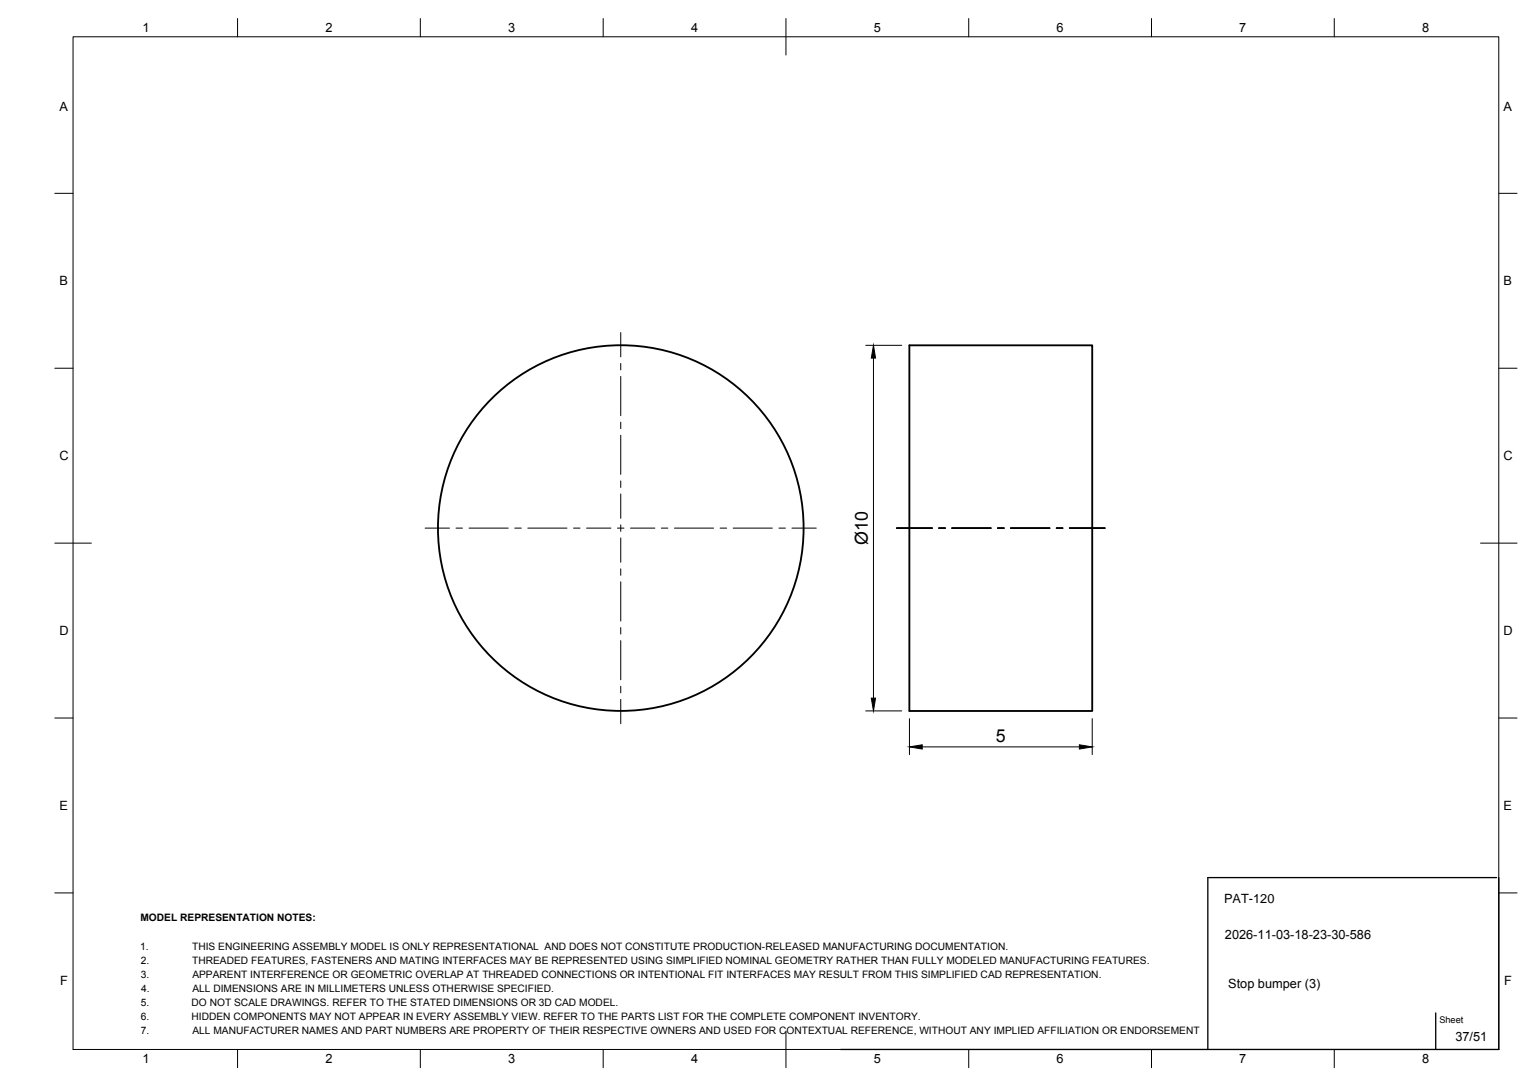
ISO-10303-21;
HEADER;
/* Generated by software containing ST-Developer
 * from STEP Tools, Inc. (www.steptools.com) 
 */

FILE_DESCRIPTION(
/* description */ ('Vibration shaker table dummy'),
/* implementation_level */ '2;1');

FILE_NAME(
/* name */ 'Stop bumper (3).step',
/* time_stamp */ '2026-10-27T10:55:14-07:00',
/* author */ (''),
/* organization */ (''),
/* preprocessor_version */ 'ST-DEVELOPER v20.2',
/* originating_system */ 'Autodesk Translation Framework v15.17.0.0',
/* authorisation */ '');

FILE_SCHEMA (('AUTOMOTIVE_DESIGN { 1 0 10303 214 3 1 1 }'));
ENDSEC;

DATA;
#10=MECHANICAL_DESIGN_GEOMETRIC_PRESENTATION_REPRESENTATION('',(#718),#22394);
#626=SHAPE_REPRESENTATION_RELATIONSHIP('SRR','None',#22672,#672);
#672=ADVANCED_BREP_SHAPE_REPRESENTATION('',(#764),#22378);
#718=STYLED_ITEM('',(#22975),#764);
#764=MANIFOLD_SOLID_BREP('Body1',#9236);
#1230=PLANE('',#10337);
#1231=PLANE('',#10338);
#1630=FACE_OUTER_BOUND('',#2300,.T.);
#1631=FACE_OUTER_BOUND('',#2301,.T.);
#1632=FACE_OUTER_BOUND('',#2302,.T.);
#2300=EDGE_LOOP('',(#7488,#7489,#7490,#7491));
#2301=EDGE_LOOP('',(#7492));
#2302=EDGE_LOOP('',(#7493));
#2985=LINE('',#21090,#3604);
#3604=VECTOR('',#12465,0.5);
#4114=CIRCLE('',#10335,0.5);
#4115=CIRCLE('',#10336,0.5);
#4781=VERTEX_POINT('',#21087);
#4782=VERTEX_POINT('',#21089);
#5737=EDGE_CURVE('',#4781,#4781,#4114,.T.);
#5738=EDGE_CURVE('',#4781,#4782,#2985,.T.);
#5739=EDGE_CURVE('',#4782,#4782,#4115,.T.);
#7488=ORIENTED_EDGE('',*,*,#5737,.F.);
#7489=ORIENTED_EDGE('',*,*,#5738,.T.);
#7490=ORIENTED_EDGE('',*,*,#5739,.T.);
#7491=ORIENTED_EDGE('',*,*,#5738,.F.);
#7492=ORIENTED_EDGE('',*,*,#5737,.T.);
#7493=ORIENTED_EDGE('',*,*,#5739,.F.);
#8621=CYLINDRICAL_SURFACE('',#10334,0.5);
#8995=ADVANCED_FACE('',(#1630),#8621,.T.);
#8996=ADVANCED_FACE('',(#1631),#1230,.T.);
#8997=ADVANCED_FACE('',(#1632),#1231,.F.);
#9236=CLOSED_SHELL('',(#8995,#8996,#8997));
#10333=AXIS2_PLACEMENT_3D('',#21085,#12459,#12460);
#10334=AXIS2_PLACEMENT_3D('',#21086,#12461,#12462);
#10335=AXIS2_PLACEMENT_3D('',#21088,#12463,#12464);
#10336=AXIS2_PLACEMENT_3D('',#21091,#12466,#12467);
#10337=AXIS2_PLACEMENT_3D('',#21092,#12468,#12469);
#10338=AXIS2_PLACEMENT_3D('',#21093,#12470,#12471);
#12459=DIRECTION('axis',(0.,0.,1.));
#12460=DIRECTION('refdir',(1.,0.,0.));
#12461=DIRECTION('center_axis',(0.,0.,1.));
#12462=DIRECTION('ref_axis',(1.,0.,0.));
#12463=DIRECTION('center_axis',(0.,0.,1.));
#12464=DIRECTION('ref_axis',(1.,0.,0.));
#12465=DIRECTION('',(0.,0.,-1.));
#12466=DIRECTION('center_axis',(0.,0.,1.));
#12467=DIRECTION('ref_axis',(1.,0.,0.));
#12468=DIRECTION('center_axis',(0.,0.,1.));
#12469=DIRECTION('ref_axis',(1.,0.,0.));
#12470=DIRECTION('center_axis',(0.,0.,1.));
#12471=DIRECTION('ref_axis',(1.,0.,0.));
#21085=CARTESIAN_POINT('',(0.,0.,0.));
#21086=CARTESIAN_POINT('Origin',(0.,6.,17.3));
#21087=CARTESIAN_POINT('',(-0.5,6.,17.8));
#21088=CARTESIAN_POINT('Origin',(0.,6.,17.8));
#21089=CARTESIAN_POINT('',(-0.5,6.,17.3));
#21090=CARTESIAN_POINT('',(-0.5,6.,17.3));
#21091=CARTESIAN_POINT('Origin',(0.,6.,17.3));
#21092=CARTESIAN_POINT('Origin',(0.,6.,17.8));
#21093=CARTESIAN_POINT('Origin',(0.,6.,17.3));
#22327=UNCERTAINTY_MEASURE_WITH_UNIT(LENGTH_MEASURE(0.001),#22395,
'DISTANCE_ACCURACY_VALUE',
'Maximum model space distance between geometric entities at asserted c
onnectivities');
#22343=UNCERTAINTY_MEASURE_WITH_UNIT(LENGTH_MEASURE(0.001),#22395,
'DISTANCE_ACCURACY_VALUE',
'Maximum model space distance between geometric entities at asserted c
onnectivities');
#22378=(
GEOMETRIC_REPRESENTATION_CONTEXT(3)
GLOBAL_UNCERTAINTY_ASSIGNED_CONTEXT((#22327))
GLOBAL_UNIT_ASSIGNED_CONTEXT((#22395,#22397,#22398))
REPRESENTATION_CONTEXT('','3D')
);
#22394=(
GEOMETRIC_REPRESENTATION_CONTEXT(3)
GLOBAL_UNCERTAINTY_ASSIGNED_CONTEXT((#22343))
GLOBAL_UNIT_ASSIGNED_CONTEXT((#22395,#22397,#22398))
REPRESENTATION_CONTEXT('','3D')
);
#22395=(
LENGTH_UNIT()
NAMED_UNIT(*)
SI_UNIT(.CENTI.,.METRE.)
);
#22397=(
NAMED_UNIT(*)
PLANE_ANGLE_UNIT()
SI_UNIT($,.RADIAN.)
);
#22398=(
NAMED_UNIT(*)
SI_UNIT($,.STERADIAN.)
SOLID_ANGLE_UNIT()
);
#22433=SHAPE_DEFINITION_REPRESENTATION(#22483,#22672);
#22483=PRODUCT_DEFINITION_SHAPE('',$,#22723);
#22672=SHAPE_REPRESENTATION('',(#10333),#22378);
#22688=PRODUCT_DEFINITION_CONTEXT('part definition',#22840,'design');
#22723=PRODUCT_DEFINITION('Stop bumper (3)','Stop bumper (3)',#22773,#22688);
#22773=PRODUCT_DEFINITION_FORMATION('',$,#22876);
#22840=APPLICATION_CONTEXT(
'Core Data for Automotive Mechanical Design Process');
#22841=PRODUCT_CONTEXT('part definition',#22840,'mechanical');
#22876=PRODUCT('Stop bumper (3)','Stop bumper (3)','Stop bumper (3)',(#22841));
#22969=COLOUR_RGB('Off White',0.89,0.88,0.83);
#22970=FILL_AREA_STYLE_COLOUR('',#22969);
#22971=FILL_AREA_STYLE('',(#22970));
#22972=SURFACE_STYLE_FILL_AREA(#22971);
#22973=SURFACE_SIDE_STYLE('',(#22972));
#22974=SURFACE_STYLE_USAGE(.BOTH.,#22973);
#22975=PRESENTATION_STYLE_ASSIGNMENT((#22974));
ENDSEC;
END-ISO-10303-21;
